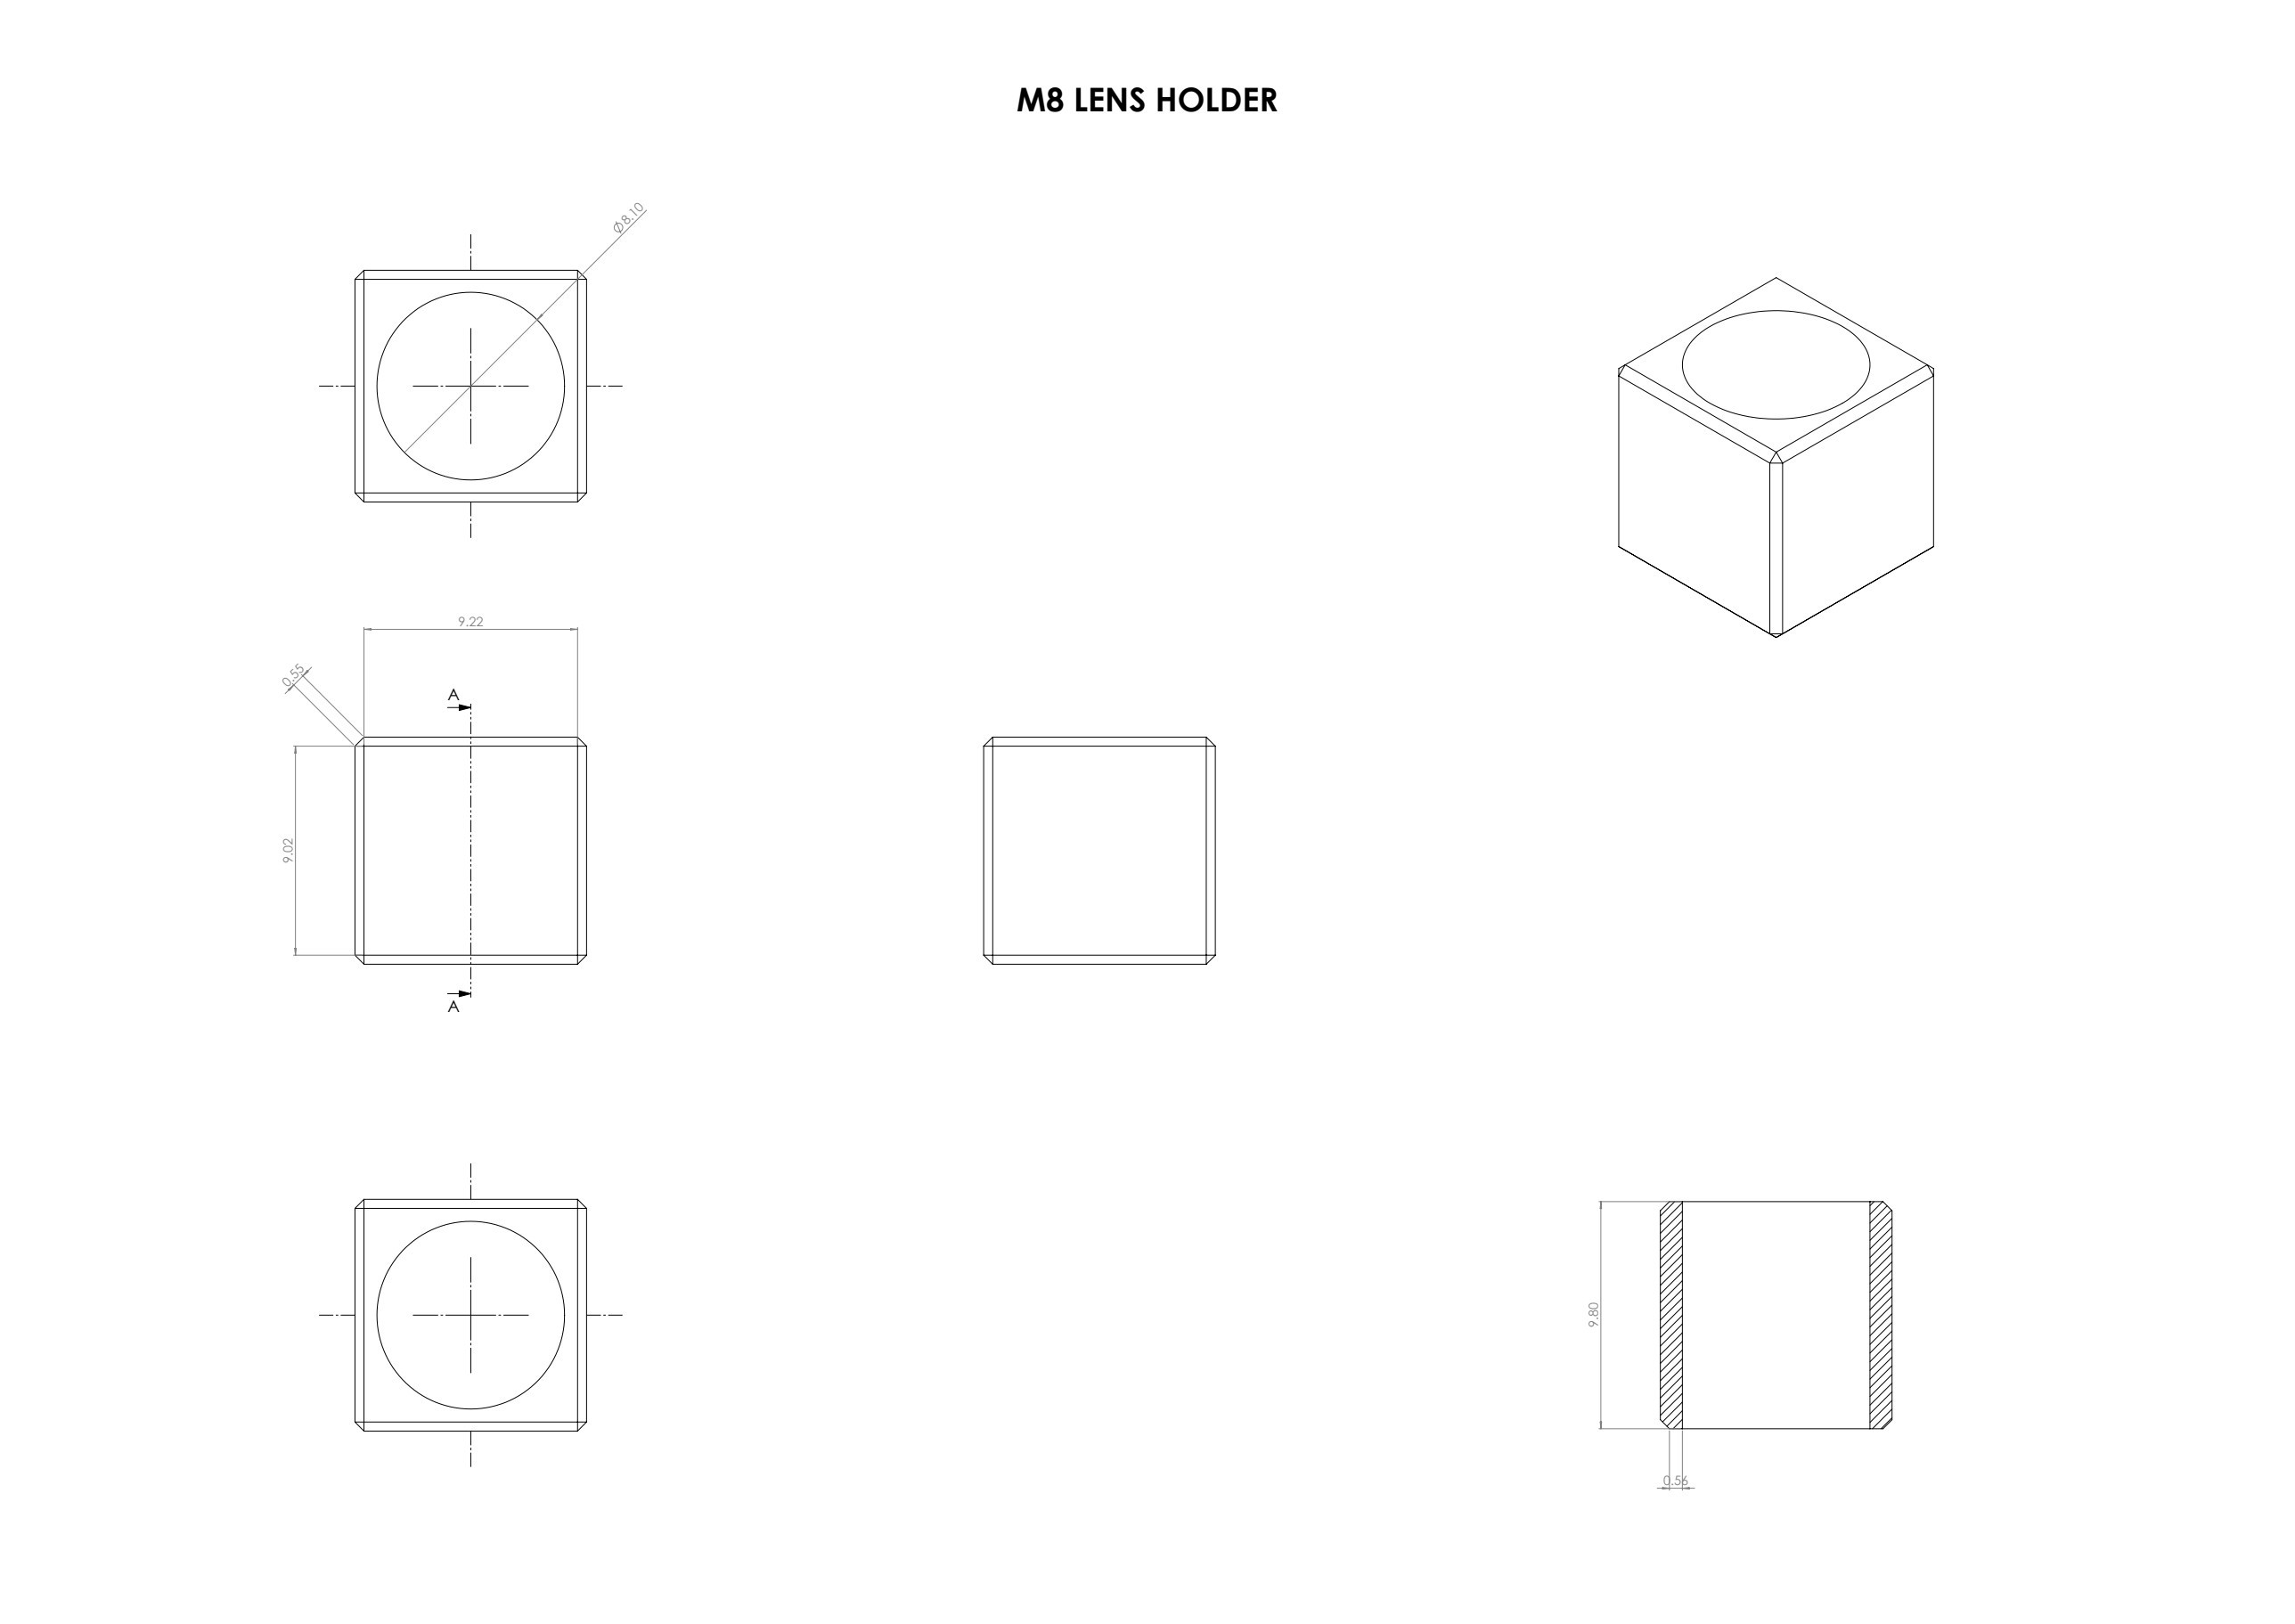
ISO-10303-21;
HEADER;
/* Generated by software containing ST-Developer
 * from STEP Tools, Inc. (www.steptools.com) 
 */

FILE_DESCRIPTION(
/* description */ (''),
/* implementation_level */ '2;1');

FILE_NAME(
/* name */ '06_M8_Lens_Holder.step',
/* time_stamp */ '2026-10-21T02:01:14-07:00',
/* author */ (''),
/* organization */ (''),
/* preprocessor_version */ 'ST-DEVELOPER v20.2',
/* originating_system */ 'Autodesk Translation Framework v15.15.0.0',
/* authorisation */ '');

FILE_SCHEMA (('AUTOMOTIVE_DESIGN { 1 0 10303 214 3 1 1 }'));
ENDSEC;

DATA;
#10=MECHANICAL_DESIGN_GEOMETRIC_PRESENTATION_REPRESENTATION('',(#619),#37181);
#593=SHAPE_REPRESENTATION_RELATIONSHIP('SRR','None',#37243,#606);
#606=ADVANCED_BREP_SHAPE_REPRESENTATION('',(#632),#37173);
#619=STYLED_ITEM('',(#37366),#632);
#632=MANIFOLD_SOLID_BREP('Body1',#14781);
#674=FACE_BOUND('',#2614,.T.);
#675=FACE_BOUND('',#2617,.T.);
#726=CYLINDRICAL_SURFACE('',#15454,4.05);
#1094=CIRCLE('',#15449,4.05);
#1095=CIRCLE('',#15452,4.05);
#1717=FACE_OUTER_BOUND('',#2591,.T.);
#1718=FACE_OUTER_BOUND('',#2592,.T.);
#1719=FACE_OUTER_BOUND('',#2593,.T.);
#1720=FACE_OUTER_BOUND('',#2594,.T.);
#1721=FACE_OUTER_BOUND('',#2595,.T.);
#1722=FACE_OUTER_BOUND('',#2596,.T.);
#1723=FACE_OUTER_BOUND('',#2597,.T.);
#1724=FACE_OUTER_BOUND('',#2598,.T.);
#1725=FACE_OUTER_BOUND('',#2599,.T.);
#1726=FACE_OUTER_BOUND('',#2600,.T.);
#1727=FACE_OUTER_BOUND('',#2601,.T.);
#1728=FACE_OUTER_BOUND('',#2602,.T.);
#1729=FACE_OUTER_BOUND('',#2603,.T.);
#1730=FACE_OUTER_BOUND('',#2604,.T.);
#1731=FACE_OUTER_BOUND('',#2605,.T.);
#1732=FACE_OUTER_BOUND('',#2606,.T.);
#1733=FACE_OUTER_BOUND('',#2607,.T.);
#1734=FACE_OUTER_BOUND('',#2608,.T.);
#1735=FACE_OUTER_BOUND('',#2609,.T.);
#1736=FACE_OUTER_BOUND('',#2610,.T.);
#1737=FACE_OUTER_BOUND('',#2611,.T.);
#1738=FACE_OUTER_BOUND('',#2612,.T.);
#1739=FACE_OUTER_BOUND('',#2613,.T.);
#1740=FACE_OUTER_BOUND('',#2615,.T.);
#1741=FACE_OUTER_BOUND('',#2616,.T.);
#1742=FACE_OUTER_BOUND('',#2618,.T.);
#1743=FACE_OUTER_BOUND('',#2619,.T.);
#2591=EDGE_LOOP('',(#10837,#10838,#10839));
#2592=EDGE_LOOP('',(#10840,#10841,#10842));
#2593=EDGE_LOOP('',(#10843,#10844,#10845));
#2594=EDGE_LOOP('',(#10846,#10847,#10848));
#2595=EDGE_LOOP('',(#10849,#10850,#10851));
#2596=EDGE_LOOP('',(#10852,#10853,#10854));
#2597=EDGE_LOOP('',(#10855,#10856,#10857));
#2598=EDGE_LOOP('',(#10858,#10859,#10860,#10861));
#2599=EDGE_LOOP('',(#10862,#10863,#10864));
#2600=EDGE_LOOP('',(#10865,#10866,#10867,#10868));
#2601=EDGE_LOOP('',(#10869,#10870,#10871,#10872));
#2602=EDGE_LOOP('',(#10873,#10874,#10875,#10876));
#2603=EDGE_LOOP('',(#10877,#10878,#10879,#10880));
#2604=EDGE_LOOP('',(#10881,#10882,#10883,#10884));
#2605=EDGE_LOOP('',(#10885,#10886,#10887,#10888));
#2606=EDGE_LOOP('',(#10889,#10890,#10891,#10892));
#2607=EDGE_LOOP('',(#10893,#10894,#10895,#10896));
#2608=EDGE_LOOP('',(#10897,#10898,#10899,#10900));
#2609=EDGE_LOOP('',(#10901,#10902,#10903,#10904));
#2610=EDGE_LOOP('',(#10905,#10906,#10907,#10908));
#2611=EDGE_LOOP('',(#10909,#10910,#10911,#10912));
#2612=EDGE_LOOP('',(#10913,#10914,#10915,#10916));
#2613=EDGE_LOOP('',(#10917,#10918,#10919,#10920));
#2614=EDGE_LOOP('',(#10921));
#2615=EDGE_LOOP('',(#10922,#10923,#10924,#10925));
#2616=EDGE_LOOP('',(#10926,#10927,#10928,#10929));
#2617=EDGE_LOOP('',(#10930));
#2618=EDGE_LOOP('',(#10931,#10932,#10933,#10934));
#2619=EDGE_LOOP('',(#10935,#10936,#10937,#10938));
#3832=LINE('',#21697,#5071);
#3833=LINE('',#21699,#5072);
#3834=LINE('',#21700,#5073);
#3835=LINE('',#21704,#5074);
#3836=LINE('',#21706,#5075);
#3837=LINE('',#21707,#5076);
#3838=LINE('',#21711,#5077);
#3839=LINE('',#21713,#5078);
#3840=LINE('',#21714,#5079);
#3841=LINE('',#21718,#5080);
#3842=LINE('',#21720,#5081);
#3843=LINE('',#21721,#5082);
#3844=LINE('',#21725,#5083);
#3845=LINE('',#21727,#5084);
#3846=LINE('',#21728,#5085);
#3847=LINE('',#21732,#5086);
#3848=LINE('',#21734,#5087);
#3849=LINE('',#21735,#5088);
#3850=LINE('',#21739,#5089);
#3851=LINE('',#21741,#5090);
#3852=LINE('',#21742,#5091);
#3853=LINE('',#21744,#5092);
#3854=LINE('',#21745,#5093);
#3855=LINE('',#21749,#5094);
#3856=LINE('',#21751,#5095);
#3857=LINE('',#21752,#5096);
#3858=LINE('',#21754,#5097);
#3859=LINE('',#21755,#5098);
#3860=LINE('',#21757,#5099);
#3861=LINE('',#21758,#5100);
#3862=LINE('',#21760,#5101);
#3863=LINE('',#21761,#5102);
#3864=LINE('',#21763,#5103);
#3865=LINE('',#21764,#5104);
#3866=LINE('',#21766,#5105);
#3867=LINE('',#21767,#5106);
#3868=LINE('',#21769,#5107);
#3869=LINE('',#21770,#5108);
#3870=LINE('',#21772,#5109);
#3871=LINE('',#21773,#5110);
#3872=LINE('',#21775,#5111);
#3873=LINE('',#21776,#5112);
#3874=LINE('',#21778,#5113);
#3875=LINE('',#21779,#5114);
#3876=LINE('',#21781,#5115);
#3877=LINE('',#21782,#5116);
#3878=LINE('',#21784,#5117);
#3879=LINE('',#21785,#5118);
#3880=LINE('',#21797,#5119);
#5071=VECTOR('',#17742,10.);
#5072=VECTOR('',#17743,10.);
#5073=VECTOR('',#17744,10.);
#5074=VECTOR('',#17747,10.);
#5075=VECTOR('',#17748,10.);
#5076=VECTOR('',#17749,10.);
#5077=VECTOR('',#17752,10.);
#5078=VECTOR('',#17753,10.);
#5079=VECTOR('',#17754,10.);
#5080=VECTOR('',#17757,10.);
#5081=VECTOR('',#17758,10.);
#5082=VECTOR('',#17759,10.);
#5083=VECTOR('',#17762,10.);
#5084=VECTOR('',#17763,10.);
#5085=VECTOR('',#17764,10.);
#5086=VECTOR('',#17767,10.);
#5087=VECTOR('',#17768,10.);
#5088=VECTOR('',#17769,10.);
#5089=VECTOR('',#17772,10.);
#5090=VECTOR('',#17773,10.);
#5091=VECTOR('',#17774,10.);
#5092=VECTOR('',#17777,10.);
#5093=VECTOR('',#17778,10.);
#5094=VECTOR('',#17781,10.);
#5095=VECTOR('',#17782,10.);
#5096=VECTOR('',#17783,10.);
#5097=VECTOR('',#17786,10.);
#5098=VECTOR('',#17787,10.);
#5099=VECTOR('',#17790,10.);
#5100=VECTOR('',#17791,10.);
#5101=VECTOR('',#17794,10.);
#5102=VECTOR('',#17795,10.);
#5103=VECTOR('',#17798,10.);
#5104=VECTOR('',#17799,10.);
#5105=VECTOR('',#17802,10.);
#5106=VECTOR('',#17803,10.);
#5107=VECTOR('',#17806,10.);
#5108=VECTOR('',#17807,10.);
#5109=VECTOR('',#17810,10.);
#5110=VECTOR('',#17811,10.);
#5111=VECTOR('',#17814,10.);
#5112=VECTOR('',#17815,10.);
#5113=VECTOR('',#17818,10.);
#5114=VECTOR('',#17819,10.);
#5115=VECTOR('',#17822,10.);
#5116=VECTOR('',#17823,10.);
#5117=VECTOR('',#17826,10.);
#5118=VECTOR('',#17827,10.);
#5119=VECTOR('',#17846,4.05);
#6183=VERTEX_POINT('',#21695);
#6184=VERTEX_POINT('',#21696);
#6185=VERTEX_POINT('',#21698);
#6186=VERTEX_POINT('',#21702);
#6187=VERTEX_POINT('',#21703);
#6188=VERTEX_POINT('',#21705);
#6189=VERTEX_POINT('',#21709);
#6190=VERTEX_POINT('',#21710);
#6191=VERTEX_POINT('',#21712);
#6192=VERTEX_POINT('',#21716);
#6193=VERTEX_POINT('',#21717);
#6194=VERTEX_POINT('',#21719);
#6195=VERTEX_POINT('',#21723);
#6196=VERTEX_POINT('',#21724);
#6197=VERTEX_POINT('',#21726);
#6198=VERTEX_POINT('',#21730);
#6199=VERTEX_POINT('',#21731);
#6200=VERTEX_POINT('',#21733);
#6201=VERTEX_POINT('',#21737);
#6202=VERTEX_POINT('',#21738);
#6203=VERTEX_POINT('',#21740);
#6204=VERTEX_POINT('',#21747);
#6205=VERTEX_POINT('',#21748);
#6206=VERTEX_POINT('',#21750);
#6207=VERTEX_POINT('',#21789);
#6208=VERTEX_POINT('',#21793);
#7860=EDGE_CURVE('',#6183,#6184,#3832,.T.);
#7861=EDGE_CURVE('',#6185,#6183,#3833,.T.);
#7862=EDGE_CURVE('',#6184,#6185,#3834,.T.);
#7863=EDGE_CURVE('',#6186,#6187,#3835,.T.);
#7864=EDGE_CURVE('',#6188,#6186,#3836,.T.);
#7865=EDGE_CURVE('',#6187,#6188,#3837,.T.);
#7866=EDGE_CURVE('',#6189,#6190,#3838,.T.);
#7867=EDGE_CURVE('',#6191,#6189,#3839,.T.);
#7868=EDGE_CURVE('',#6190,#6191,#3840,.T.);
#7869=EDGE_CURVE('',#6192,#6193,#3841,.T.);
#7870=EDGE_CURVE('',#6194,#6192,#3842,.T.);
#7871=EDGE_CURVE('',#6193,#6194,#3843,.T.);
#7872=EDGE_CURVE('',#6195,#6196,#3844,.T.);
#7873=EDGE_CURVE('',#6197,#6195,#3845,.T.);
#7874=EDGE_CURVE('',#6196,#6197,#3846,.T.);
#7875=EDGE_CURVE('',#6198,#6199,#3847,.T.);
#7876=EDGE_CURVE('',#6200,#6198,#3848,.T.);
#7877=EDGE_CURVE('',#6199,#6200,#3849,.T.);
#7878=EDGE_CURVE('',#6201,#6202,#3850,.T.);
#7879=EDGE_CURVE('',#6203,#6201,#3851,.T.);
#7880=EDGE_CURVE('',#6202,#6203,#3852,.T.);
#7881=EDGE_CURVE('',#6191,#6203,#3853,.T.);
#7882=EDGE_CURVE('',#6201,#6190,#3854,.T.);
#7883=EDGE_CURVE('',#6204,#6205,#3855,.T.);
#7884=EDGE_CURVE('',#6206,#6204,#3856,.T.);
#7885=EDGE_CURVE('',#6205,#6206,#3857,.T.);
#7886=EDGE_CURVE('',#6204,#6197,#3858,.T.);
#7887=EDGE_CURVE('',#6195,#6206,#3859,.T.);
#7888=EDGE_CURVE('',#6198,#6205,#3860,.T.);
#7889=EDGE_CURVE('',#6206,#6200,#3861,.T.);
#7890=EDGE_CURVE('',#6203,#6204,#3862,.T.);
#7891=EDGE_CURVE('',#6205,#6202,#3863,.T.);
#7892=EDGE_CURVE('',#6192,#6201,#3864,.T.);
#7893=EDGE_CURVE('',#6202,#6194,#3865,.T.);
#7894=EDGE_CURVE('',#6187,#6199,#3866,.T.);
#7895=EDGE_CURVE('',#6200,#6186,#3867,.T.);
#7896=EDGE_CURVE('',#6199,#6193,#3868,.T.);
#7897=EDGE_CURVE('',#6194,#6198,#3869,.T.);
#7898=EDGE_CURVE('',#6197,#6191,#3870,.T.);
#7899=EDGE_CURVE('',#6189,#6196,#3871,.T.);
#7900=EDGE_CURVE('',#6186,#6195,#3872,.T.);
#7901=EDGE_CURVE('',#6196,#6188,#3873,.T.);
#7902=EDGE_CURVE('',#6193,#6184,#3874,.T.);
#7903=EDGE_CURVE('',#6185,#6192,#3875,.T.);
#7904=EDGE_CURVE('',#6183,#6189,#3876,.T.);
#7905=EDGE_CURVE('',#6190,#6185,#3877,.T.);
#7906=EDGE_CURVE('',#6184,#6187,#3878,.T.);
#7907=EDGE_CURVE('',#6188,#6183,#3879,.T.);
#7908=EDGE_CURVE('',#6207,#6207,#1094,.T.);
#7909=EDGE_CURVE('',#6208,#6208,#1095,.T.);
#7910=EDGE_CURVE('',#6208,#6207,#3880,.T.);
#10837=ORIENTED_EDGE('',*,*,#7860,.F.);
#10838=ORIENTED_EDGE('',*,*,#7861,.F.);
#10839=ORIENTED_EDGE('',*,*,#7862,.F.);
#10840=ORIENTED_EDGE('',*,*,#7863,.F.);
#10841=ORIENTED_EDGE('',*,*,#7864,.F.);
#10842=ORIENTED_EDGE('',*,*,#7865,.F.);
#10843=ORIENTED_EDGE('',*,*,#7866,.F.);
#10844=ORIENTED_EDGE('',*,*,#7867,.F.);
#10845=ORIENTED_EDGE('',*,*,#7868,.F.);
#10846=ORIENTED_EDGE('',*,*,#7869,.F.);
#10847=ORIENTED_EDGE('',*,*,#7870,.F.);
#10848=ORIENTED_EDGE('',*,*,#7871,.F.);
#10849=ORIENTED_EDGE('',*,*,#7872,.F.);
#10850=ORIENTED_EDGE('',*,*,#7873,.F.);
#10851=ORIENTED_EDGE('',*,*,#7874,.F.);
#10852=ORIENTED_EDGE('',*,*,#7875,.F.);
#10853=ORIENTED_EDGE('',*,*,#7876,.F.);
#10854=ORIENTED_EDGE('',*,*,#7877,.F.);
#10855=ORIENTED_EDGE('',*,*,#7878,.F.);
#10856=ORIENTED_EDGE('',*,*,#7879,.F.);
#10857=ORIENTED_EDGE('',*,*,#7880,.F.);
#10858=ORIENTED_EDGE('',*,*,#7868,.T.);
#10859=ORIENTED_EDGE('',*,*,#7881,.T.);
#10860=ORIENTED_EDGE('',*,*,#7879,.T.);
#10861=ORIENTED_EDGE('',*,*,#7882,.T.);
#10862=ORIENTED_EDGE('',*,*,#7883,.F.);
#10863=ORIENTED_EDGE('',*,*,#7884,.F.);
#10864=ORIENTED_EDGE('',*,*,#7885,.F.);
#10865=ORIENTED_EDGE('',*,*,#7884,.T.);
#10866=ORIENTED_EDGE('',*,*,#7886,.T.);
#10867=ORIENTED_EDGE('',*,*,#7873,.T.);
#10868=ORIENTED_EDGE('',*,*,#7887,.T.);
#10869=ORIENTED_EDGE('',*,*,#7876,.T.);
#10870=ORIENTED_EDGE('',*,*,#7888,.T.);
#10871=ORIENTED_EDGE('',*,*,#7885,.T.);
#10872=ORIENTED_EDGE('',*,*,#7889,.T.);
#10873=ORIENTED_EDGE('',*,*,#7880,.T.);
#10874=ORIENTED_EDGE('',*,*,#7890,.T.);
#10875=ORIENTED_EDGE('',*,*,#7883,.T.);
#10876=ORIENTED_EDGE('',*,*,#7891,.T.);
#10877=ORIENTED_EDGE('',*,*,#7870,.T.);
#10878=ORIENTED_EDGE('',*,*,#7892,.T.);
#10879=ORIENTED_EDGE('',*,*,#7878,.T.);
#10880=ORIENTED_EDGE('',*,*,#7893,.T.);
#10881=ORIENTED_EDGE('',*,*,#7863,.T.);
#10882=ORIENTED_EDGE('',*,*,#7894,.T.);
#10883=ORIENTED_EDGE('',*,*,#7877,.T.);
#10884=ORIENTED_EDGE('',*,*,#7895,.T.);
#10885=ORIENTED_EDGE('',*,*,#7875,.T.);
#10886=ORIENTED_EDGE('',*,*,#7896,.T.);
#10887=ORIENTED_EDGE('',*,*,#7871,.T.);
#10888=ORIENTED_EDGE('',*,*,#7897,.T.);
#10889=ORIENTED_EDGE('',*,*,#7874,.T.);
#10890=ORIENTED_EDGE('',*,*,#7898,.T.);
#10891=ORIENTED_EDGE('',*,*,#7867,.T.);
#10892=ORIENTED_EDGE('',*,*,#7899,.T.);
#10893=ORIENTED_EDGE('',*,*,#7864,.T.);
#10894=ORIENTED_EDGE('',*,*,#7900,.T.);
#10895=ORIENTED_EDGE('',*,*,#7872,.T.);
#10896=ORIENTED_EDGE('',*,*,#7901,.T.);
#10897=ORIENTED_EDGE('',*,*,#7869,.T.);
#10898=ORIENTED_EDGE('',*,*,#7902,.T.);
#10899=ORIENTED_EDGE('',*,*,#7862,.T.);
#10900=ORIENTED_EDGE('',*,*,#7903,.T.);
#10901=ORIENTED_EDGE('',*,*,#7861,.T.);
#10902=ORIENTED_EDGE('',*,*,#7904,.T.);
#10903=ORIENTED_EDGE('',*,*,#7866,.T.);
#10904=ORIENTED_EDGE('',*,*,#7905,.T.);
#10905=ORIENTED_EDGE('',*,*,#7860,.T.);
#10906=ORIENTED_EDGE('',*,*,#7906,.T.);
#10907=ORIENTED_EDGE('',*,*,#7865,.T.);
#10908=ORIENTED_EDGE('',*,*,#7907,.T.);
#10909=ORIENTED_EDGE('',*,*,#7882,.F.);
#10910=ORIENTED_EDGE('',*,*,#7892,.F.);
#10911=ORIENTED_EDGE('',*,*,#7903,.F.);
#10912=ORIENTED_EDGE('',*,*,#7905,.F.);
#10913=ORIENTED_EDGE('',*,*,#7887,.F.);
#10914=ORIENTED_EDGE('',*,*,#7900,.F.);
#10915=ORIENTED_EDGE('',*,*,#7895,.F.);
#10916=ORIENTED_EDGE('',*,*,#7889,.F.);
#10917=ORIENTED_EDGE('',*,*,#7886,.F.);
#10918=ORIENTED_EDGE('',*,*,#7890,.F.);
#10919=ORIENTED_EDGE('',*,*,#7881,.F.);
#10920=ORIENTED_EDGE('',*,*,#7898,.F.);
#10921=ORIENTED_EDGE('',*,*,#7908,.T.);
#10922=ORIENTED_EDGE('',*,*,#7888,.F.);
#10923=ORIENTED_EDGE('',*,*,#7897,.F.);
#10924=ORIENTED_EDGE('',*,*,#7893,.F.);
#10925=ORIENTED_EDGE('',*,*,#7891,.F.);
#10926=ORIENTED_EDGE('',*,*,#7894,.F.);
#10927=ORIENTED_EDGE('',*,*,#7906,.F.);
#10928=ORIENTED_EDGE('',*,*,#7902,.F.);
#10929=ORIENTED_EDGE('',*,*,#7896,.F.);
#10930=ORIENTED_EDGE('',*,*,#7909,.T.);
#10931=ORIENTED_EDGE('',*,*,#7899,.F.);
#10932=ORIENTED_EDGE('',*,*,#7904,.F.);
#10933=ORIENTED_EDGE('',*,*,#7907,.F.);
#10934=ORIENTED_EDGE('',*,*,#7901,.F.);
#10935=ORIENTED_EDGE('',*,*,#7909,.F.);
#10936=ORIENTED_EDGE('',*,*,#7910,.T.);
#10937=ORIENTED_EDGE('',*,*,#7908,.F.);
#10938=ORIENTED_EDGE('',*,*,#7910,.F.);
#13700=PLANE('',#15426);
#13701=PLANE('',#15427);
#13702=PLANE('',#15428);
#13703=PLANE('',#15429);
#13704=PLANE('',#15430);
#13705=PLANE('',#15431);
#13706=PLANE('',#15432);
#13707=PLANE('',#15433);
#13708=PLANE('',#15434);
#13709=PLANE('',#15435);
#13710=PLANE('',#15436);
#13711=PLANE('',#15437);
#13712=PLANE('',#15438);
#13713=PLANE('',#15439);
#13714=PLANE('',#15440);
#13715=PLANE('',#15441);
#13716=PLANE('',#15442);
#13717=PLANE('',#15443);
#13718=PLANE('',#15444);
#13719=PLANE('',#15445);
#13720=PLANE('',#15446);
#13721=PLANE('',#15447);
#13722=PLANE('',#15448);
#13723=PLANE('',#15450);
#13724=PLANE('',#15451);
#13725=PLANE('',#15453);
#14285=ADVANCED_FACE('',(#1717),#13700,.T.);
#14286=ADVANCED_FACE('',(#1718),#13701,.T.);
#14287=ADVANCED_FACE('',(#1719),#13702,.T.);
#14288=ADVANCED_FACE('',(#1720),#13703,.T.);
#14289=ADVANCED_FACE('',(#1721),#13704,.T.);
#14290=ADVANCED_FACE('',(#1722),#13705,.T.);
#14291=ADVANCED_FACE('',(#1723),#13706,.T.);
#14292=ADVANCED_FACE('',(#1724),#13707,.T.);
#14293=ADVANCED_FACE('',(#1725),#13708,.T.);
#14294=ADVANCED_FACE('',(#1726),#13709,.T.);
#14295=ADVANCED_FACE('',(#1727),#13710,.T.);
#14296=ADVANCED_FACE('',(#1728),#13711,.T.);
#14297=ADVANCED_FACE('',(#1729),#13712,.T.);
#14298=ADVANCED_FACE('',(#1730),#13713,.T.);
#14299=ADVANCED_FACE('',(#1731),#13714,.T.);
#14300=ADVANCED_FACE('',(#1732),#13715,.T.);
#14301=ADVANCED_FACE('',(#1733),#13716,.T.);
#14302=ADVANCED_FACE('',(#1734),#13717,.T.);
#14303=ADVANCED_FACE('',(#1735),#13718,.T.);
#14304=ADVANCED_FACE('',(#1736),#13719,.T.);
#14305=ADVANCED_FACE('',(#1737),#13720,.T.);
#14306=ADVANCED_FACE('',(#1738),#13721,.T.);
#14307=ADVANCED_FACE('',(#1739,#674),#13722,.F.);
#14308=ADVANCED_FACE('',(#1740),#13723,.T.);
#14309=ADVANCED_FACE('',(#1741,#675),#13724,.T.);
#14310=ADVANCED_FACE('',(#1742),#13725,.T.);
#14311=ADVANCED_FACE('',(#1743),#726,.F.);
#14781=CLOSED_SHELL('',(#14285,#14286,#14287,#14288,#14289,#14290,#14291,
#14292,#14293,#14294,#14295,#14296,#14297,#14298,#14299,#14300,#14301,#14302,
#14303,#14304,#14305,#14306,#14307,#14308,#14309,#14310,#14311));
#15425=AXIS2_PLACEMENT_3D('',#21693,#17738,#17739);
#15426=AXIS2_PLACEMENT_3D('',#21694,#17740,#17741);
#15427=AXIS2_PLACEMENT_3D('',#21701,#17745,#17746);
#15428=AXIS2_PLACEMENT_3D('',#21708,#17750,#17751);
#15429=AXIS2_PLACEMENT_3D('',#21715,#17755,#17756);
#15430=AXIS2_PLACEMENT_3D('',#21722,#17760,#17761);
#15431=AXIS2_PLACEMENT_3D('',#21729,#17765,#17766);
#15432=AXIS2_PLACEMENT_3D('',#21736,#17770,#17771);
#15433=AXIS2_PLACEMENT_3D('',#21743,#17775,#17776);
#15434=AXIS2_PLACEMENT_3D('',#21746,#17779,#17780);
#15435=AXIS2_PLACEMENT_3D('',#21753,#17784,#17785);
#15436=AXIS2_PLACEMENT_3D('',#21756,#17788,#17789);
#15437=AXIS2_PLACEMENT_3D('',#21759,#17792,#17793);
#15438=AXIS2_PLACEMENT_3D('',#21762,#17796,#17797);
#15439=AXIS2_PLACEMENT_3D('',#21765,#17800,#17801);
#15440=AXIS2_PLACEMENT_3D('',#21768,#17804,#17805);
#15441=AXIS2_PLACEMENT_3D('',#21771,#17808,#17809);
#15442=AXIS2_PLACEMENT_3D('',#21774,#17812,#17813);
#15443=AXIS2_PLACEMENT_3D('',#21777,#17816,#17817);
#15444=AXIS2_PLACEMENT_3D('',#21780,#17820,#17821);
#15445=AXIS2_PLACEMENT_3D('',#21783,#17824,#17825);
#15446=AXIS2_PLACEMENT_3D('',#21786,#17828,#17829);
#15447=AXIS2_PLACEMENT_3D('',#21787,#17830,#17831);
#15448=AXIS2_PLACEMENT_3D('',#21788,#17832,#17833);
#15449=AXIS2_PLACEMENT_3D('',#21790,#17834,#17835);
#15450=AXIS2_PLACEMENT_3D('',#21791,#17836,#17837);
#15451=AXIS2_PLACEMENT_3D('',#21792,#17838,#17839);
#15452=AXIS2_PLACEMENT_3D('',#21794,#17840,#17841);
#15453=AXIS2_PLACEMENT_3D('',#21795,#17842,#17843);
#15454=AXIS2_PLACEMENT_3D('',#21796,#17844,#17845);
#17738=DIRECTION('axis',(0.,0.,1.));
#17739=DIRECTION('refdir',(1.,0.,0.));
#17740=DIRECTION('center_axis',(0.577350269189623,0.577350269189625,-0.57735026918963));
#17741=DIRECTION('ref_axis',(-0.707106781186552,0.,-0.707106781186544));
#17742=DIRECTION('',(-0.707106781186548,0.707106781186546,0.));
#17743=DIRECTION('',(0.707106781186552,0.,0.707106781186543));
#17744=DIRECTION('',(0.,-0.70710678118655,-0.707106781186544));
#17745=DIRECTION('center_axis',(0.577350269189623,0.577350269189625,0.57735026918963));
#17746=DIRECTION('ref_axis',(0.707106781186552,0.,-0.707106781186543));
#17747=DIRECTION('',(0.,0.70710678118655,-0.707106781186544));
#17748=DIRECTION('',(-0.707106781186552,0.,0.707106781186543));
#17749=DIRECTION('',(0.707106781186548,-0.707106781186546,0.));
#17750=DIRECTION('center_axis',(0.577350269189624,-0.577350269189624,-0.57735026918963));
#17751=DIRECTION('ref_axis',(-0.707106781186552,0.,-0.707106781186544));
#17752=DIRECTION('',(-0.707106781186552,0.,-0.707106781186543));
#17753=DIRECTION('',(0.707106781186547,0.707106781186547,0.));
#17754=DIRECTION('',(0.,-0.707106781186552,0.707106781186543));
#17755=DIRECTION('center_axis',(-0.577350269189625,0.577350269189624,-0.577350269189629));
#17756=DIRECTION('ref_axis',(-0.70710678118655,0.,0.707106781186545));
#17757=DIRECTION('',(0.,0.70710678118655,0.707106781186544));
#17758=DIRECTION('',(0.70710678118655,0.,-0.707106781186545));
#17759=DIRECTION('',(-0.707106781186546,-0.707106781186549,0.));
#17760=DIRECTION('center_axis',(0.577350269189624,-0.577350269189624,0.57735026918963));
#17761=DIRECTION('ref_axis',(0.707106781186552,0.,-0.707106781186544));
#17762=DIRECTION('',(0.707106781186552,0.,-0.707106781186543));
#17763=DIRECTION('',(0.,0.707106781186552,0.707106781186543));
#17764=DIRECTION('',(-0.707106781186547,-0.707106781186547,0.));
#17765=DIRECTION('center_axis',(-0.577350269189626,0.577350269189625,0.577350269189626));
#17766=DIRECTION('ref_axis',(0.707106781186547,0.,0.707106781186547));
#17767=DIRECTION('',(0.707106781186546,0.707106781186549,0.));
#17768=DIRECTION('',(-0.707106781186547,0.,-0.707106781186547));
#17769=DIRECTION('',(-4.02587809918918E-15,-0.70710678118655,0.707106781186544));
#17770=DIRECTION('center_axis',(-0.577350269189626,-0.577350269189623,-0.577350269189629));
#17771=DIRECTION('ref_axis',(-0.70710678118655,0.,0.707106781186545));
#17772=DIRECTION('',(-0.70710678118655,0.,0.707106781186545));
#17773=DIRECTION('',(0.,0.707106781186552,-0.707106781186543));
#17774=DIRECTION('',(0.707106781186545,-0.70710678118655,0.));
#17775=DIRECTION('center_axis',(0.,-0.707106781186543,-0.707106781186552));
#17776=DIRECTION('ref_axis',(-1.,0.,0.));
#17777=DIRECTION('',(-1.,0.,0.));
#17778=DIRECTION('',(1.,0.,0.));
#17779=DIRECTION('center_axis',(-0.577350269189627,-0.577350269189624,0.577350269189627));
#17780=DIRECTION('ref_axis',(0.707106781186547,0.,0.707106781186547));
#17781=DIRECTION('',(-0.707106781186545,0.70710678118655,0.));
#17782=DIRECTION('',(4.02587809918917E-15,-0.707106781186552,-0.707106781186543));
#17783=DIRECTION('',(0.707106781186547,0.,0.707106781186547));
#17784=DIRECTION('center_axis',(0.,-0.707106781186543,0.707106781186552));
#17785=DIRECTION('ref_axis',(1.,0.,0.));
#17786=DIRECTION('',(1.,0.,0.));
#17787=DIRECTION('',(-1.,0.,0.));
#17788=DIRECTION('center_axis',(-0.707106781186548,0.,0.707106781186548));
#17789=DIRECTION('ref_axis',(0.707106781186548,0.,0.707106781186548));
#17790=DIRECTION('',(0.,-1.,0.));
#17791=DIRECTION('',(0.,1.,0.));
#17792=DIRECTION('center_axis',(-0.70710678118655,-0.707106781186546,0.));
#17793=DIRECTION('ref_axis',(0.,0.,1.));
#17794=DIRECTION('',(0.,0.,1.));
#17795=DIRECTION('',(0.,0.,-1.));
#17796=DIRECTION('center_axis',(-0.707106781186545,0.,-0.70710678118655));
#17797=DIRECTION('ref_axis',(-0.70710678118655,0.,0.707106781186545));
#17798=DIRECTION('',(0.,-1.,0.));
#17799=DIRECTION('',(0.,1.,0.));
#17800=DIRECTION('center_axis',(0.,0.707106781186545,0.707106781186551));
#17801=DIRECTION('ref_axis',(1.,0.,0.));
#17802=DIRECTION('',(-1.,0.,0.));
#17803=DIRECTION('',(1.,0.,0.));
#17804=DIRECTION('center_axis',(-0.707106781186549,0.707106781186546,0.));
#17805=DIRECTION('ref_axis',(0.,0.,1.));
#17806=DIRECTION('',(0.,0.,-1.));
#17807=DIRECTION('',(0.,0.,1.));
#17808=DIRECTION('center_axis',(0.707106781186548,-0.707106781186548,0.));
#17809=DIRECTION('ref_axis',(0.,0.,-1.));
#17810=DIRECTION('',(0.,0.,-1.));
#17811=DIRECTION('',(0.,0.,1.));
#17812=DIRECTION('center_axis',(0.707106781186543,0.,0.707106781186552));
#17813=DIRECTION('ref_axis',(0.707106781186552,0.,-0.707106781186543));
#17814=DIRECTION('',(0.,-1.,0.));
#17815=DIRECTION('',(0.,1.,0.));
#17816=DIRECTION('center_axis',(0.,0.707106781186545,-0.707106781186551));
#17817=DIRECTION('ref_axis',(-1.,0.,0.));
#17818=DIRECTION('',(1.,0.,0.));
#17819=DIRECTION('',(-1.,0.,0.));
#17820=DIRECTION('center_axis',(0.707106781186543,0.,-0.707106781186552));
#17821=DIRECTION('ref_axis',(-0.707106781186552,0.,-0.707106781186543));
#17822=DIRECTION('',(0.,-1.,0.));
#17823=DIRECTION('',(0.,1.,0.));
#17824=DIRECTION('center_axis',(0.707106781186547,0.707106781186549,0.));
#17825=DIRECTION('ref_axis',(0.,0.,-1.));
#17826=DIRECTION('',(0.,0.,1.));
#17827=DIRECTION('',(0.,0.,-1.));
#17828=DIRECTION('center_axis',(0.,0.,-1.));
#17829=DIRECTION('ref_axis',(-1.,0.,0.));
#17830=DIRECTION('center_axis',(0.,0.,1.));
#17831=DIRECTION('ref_axis',(1.,0.,0.));
#17832=DIRECTION('center_axis',(0.,1.,0.));
#17833=DIRECTION('ref_axis',(1.,0.,0.));
#17834=DIRECTION('center_axis',(0.,1.,0.));
#17835=DIRECTION('ref_axis',(1.,0.,0.));
#17836=DIRECTION('center_axis',(-1.,0.,0.));
#17837=DIRECTION('ref_axis',(0.,0.,1.));
#17838=DIRECTION('center_axis',(0.,1.,0.));
#17839=DIRECTION('ref_axis',(0.,0.,1.));
#17840=DIRECTION('center_axis',(0.,-1.,0.));
#17841=DIRECTION('ref_axis',(1.,0.,0.));
#17842=DIRECTION('center_axis',(1.,0.,0.));
#17843=DIRECTION('ref_axis',(0.,0.,-1.));
#17844=DIRECTION('center_axis',(0.,-1.,0.));
#17845=DIRECTION('ref_axis',(1.,0.,0.));
#17846=DIRECTION('',(0.,-1.,0.));
#21693=CARTESIAN_POINT('',(0.,0.,0.));
#21694=CARTESIAN_POINT('Origin',(28.61,1.61,-52.5));
#21695=CARTESIAN_POINT('',(29.,1.61,-52.11));
#21696=CARTESIAN_POINT('',(28.61,2.,-52.11));
#21697=CARTESIAN_POINT('',(29.,1.61,-52.11));
#21698=CARTESIAN_POINT('',(28.61,1.61,-52.5));
#21699=CARTESIAN_POINT('',(28.61,1.61,-52.5));
#21700=CARTESIAN_POINT('',(28.61,2.,-52.11));
#21701=CARTESIAN_POINT('Origin',(29.,1.61,-42.89));
#21702=CARTESIAN_POINT('',(28.61,1.61,-42.5));
#21703=CARTESIAN_POINT('',(28.61,2.,-42.89));
#21704=CARTESIAN_POINT('',(28.61,1.61,-42.5));
#21705=CARTESIAN_POINT('',(29.,1.61,-42.89));
#21706=CARTESIAN_POINT('',(29.,1.61,-42.89));
#21707=CARTESIAN_POINT('',(28.61,2.,-42.89));
#21708=CARTESIAN_POINT('Origin',(28.61,-7.8,-52.11));
#21709=CARTESIAN_POINT('',(29.,-7.41,-52.11));
#21710=CARTESIAN_POINT('',(28.61,-7.41,-52.5));
#21711=CARTESIAN_POINT('',(29.,-7.41,-52.11));
#21712=CARTESIAN_POINT('',(28.61,-7.8,-52.11));
#21713=CARTESIAN_POINT('',(28.61,-7.8,-52.11));
#21714=CARTESIAN_POINT('',(28.61,-7.41,-52.5));
#21715=CARTESIAN_POINT('Origin',(19.,1.61,-52.11));
#21716=CARTESIAN_POINT('',(19.39,1.61,-52.5));
#21717=CARTESIAN_POINT('',(19.39,2.,-52.11));
#21718=CARTESIAN_POINT('',(19.39,1.61,-52.5));
#21719=CARTESIAN_POINT('',(19.,1.61,-52.11));
#21720=CARTESIAN_POINT('',(19.,1.61,-52.11));
#21721=CARTESIAN_POINT('',(19.39,2.,-52.11));
#21722=CARTESIAN_POINT('Origin',(28.61,-7.8,-42.89));
#21723=CARTESIAN_POINT('',(28.61,-7.41,-42.5));
#21724=CARTESIAN_POINT('',(29.,-7.41,-42.89));
#21725=CARTESIAN_POINT('',(28.61,-7.41,-42.5));
#21726=CARTESIAN_POINT('',(28.61,-7.8,-42.89));
#21727=CARTESIAN_POINT('',(28.61,-7.8,-42.89));
#21728=CARTESIAN_POINT('',(29.,-7.41,-42.89));
#21729=CARTESIAN_POINT('Origin',(19.39,1.61,-42.5));
#21730=CARTESIAN_POINT('',(19.,1.61,-42.89));
#21731=CARTESIAN_POINT('',(19.39,2.,-42.89));
#21732=CARTESIAN_POINT('',(19.,1.61,-42.89));
#21733=CARTESIAN_POINT('',(19.39,1.61,-42.5));
#21734=CARTESIAN_POINT('',(19.39,1.61,-42.5));
#21735=CARTESIAN_POINT('',(19.39,2.,-42.89));
#21736=CARTESIAN_POINT('Origin',(19.39,-7.8,-52.11));
#21737=CARTESIAN_POINT('',(19.39,-7.41,-52.5));
#21738=CARTESIAN_POINT('',(19.,-7.41,-52.11));
#21739=CARTESIAN_POINT('',(19.39,-7.41,-52.5));
#21740=CARTESIAN_POINT('',(19.39,-7.8,-52.11));
#21741=CARTESIAN_POINT('',(19.39,-7.8,-52.11));
#21742=CARTESIAN_POINT('',(19.,-7.41,-52.11));
#21743=CARTESIAN_POINT('Origin',(26.5,-7.605,-52.305));
#21744=CARTESIAN_POINT('',(26.5,-7.8,-52.11));
#21745=CARTESIAN_POINT('',(26.5,-7.41,-52.5));
#21746=CARTESIAN_POINT('Origin',(19.39,-7.41,-42.5));
#21747=CARTESIAN_POINT('',(19.39,-7.8,-42.89));
#21748=CARTESIAN_POINT('',(19.,-7.41,-42.89));
#21749=CARTESIAN_POINT('',(19.39,-7.8,-42.89));
#21750=CARTESIAN_POINT('',(19.39,-7.41,-42.5));
#21751=CARTESIAN_POINT('',(19.39,-7.41,-42.5));
#21752=CARTESIAN_POINT('',(19.,-7.41,-42.89));
#21753=CARTESIAN_POINT('Origin',(21.5,-7.605,-42.695));
#21754=CARTESIAN_POINT('',(21.5,-7.8,-42.89));
#21755=CARTESIAN_POINT('',(21.5,-7.41,-42.5));
#21756=CARTESIAN_POINT('Origin',(19.195,-7.8,-42.695));
#21757=CARTESIAN_POINT('',(19.,-7.8,-42.89));
#21758=CARTESIAN_POINT('',(19.39,-7.8,-42.5));
#21759=CARTESIAN_POINT('Origin',(19.195,-7.605,-50.));
#21760=CARTESIAN_POINT('',(19.39,-7.8,-50.));
#21761=CARTESIAN_POINT('',(19.,-7.41,-50.));
#21762=CARTESIAN_POINT('Origin',(19.195,-7.8,-52.305));
#21763=CARTESIAN_POINT('',(19.39,-7.8,-52.5));
#21764=CARTESIAN_POINT('',(19.,-7.8,-52.11));
#21765=CARTESIAN_POINT('Origin',(21.5,1.805,-42.695));
#21766=CARTESIAN_POINT('',(21.5,2.,-42.89));
#21767=CARTESIAN_POINT('',(21.5,1.61,-42.5));
#21768=CARTESIAN_POINT('Origin',(19.195,1.805,-50.));
#21769=CARTESIAN_POINT('',(19.39,2.,-50.));
#21770=CARTESIAN_POINT('',(19.,1.61,-50.));
#21771=CARTESIAN_POINT('Origin',(28.805,-7.605,-45.));
#21772=CARTESIAN_POINT('',(28.61,-7.8,-45.));
#21773=CARTESIAN_POINT('',(29.,-7.41,-45.));
#21774=CARTESIAN_POINT('Origin',(28.805,-7.8,-42.695));
#21775=CARTESIAN_POINT('',(28.61,-7.8,-42.5));
#21776=CARTESIAN_POINT('',(29.,-7.8,-42.89));
#21777=CARTESIAN_POINT('Origin',(26.5,1.805,-52.305));
#21778=CARTESIAN_POINT('',(26.5,2.,-52.11));
#21779=CARTESIAN_POINT('',(26.5,1.61,-52.5));
#21780=CARTESIAN_POINT('Origin',(28.805,-7.8,-52.305));
#21781=CARTESIAN_POINT('',(29.,-7.8,-52.11));
#21782=CARTESIAN_POINT('',(28.61,-7.8,-52.5));
#21783=CARTESIAN_POINT('Origin',(28.805,1.805,-45.));
#21784=CARTESIAN_POINT('',(28.61,2.,-45.));
#21785=CARTESIAN_POINT('',(29.,1.61,-45.));
#21786=CARTESIAN_POINT('Origin',(29.,-7.8,-52.5));
#21787=CARTESIAN_POINT('Origin',(19.,-7.8,-42.5));
#21788=CARTESIAN_POINT('Origin',(24.,-7.8,-47.5));
#21789=CARTESIAN_POINT('',(19.95,-7.8,-47.5));
#21790=CARTESIAN_POINT('Origin',(24.,-7.8,-47.5));
#21791=CARTESIAN_POINT('Origin',(19.,-7.8,-52.5));
#21792=CARTESIAN_POINT('Origin',(24.,2.,-47.5));
#21793=CARTESIAN_POINT('',(19.95,2.,-47.5));
#21794=CARTESIAN_POINT('Origin',(24.,2.,-47.5));
#21795=CARTESIAN_POINT('Origin',(29.,-7.8,-42.5));
#21796=CARTESIAN_POINT('Origin',(24.,2.,-47.5));
#21797=CARTESIAN_POINT('',(19.95,2.,-47.5));
#37158=UNCERTAINTY_MEASURE_WITH_UNIT(LENGTH_MEASURE(0.01),#37182,
'DISTANCE_ACCURACY_VALUE',
'Maximum model space distance between geometric entities at asserted c
onnectivities');
#37166=UNCERTAINTY_MEASURE_WITH_UNIT(LENGTH_MEASURE(0.01),#37182,
'DISTANCE_ACCURACY_VALUE',
'Maximum model space distance between geometric entities at asserted c
onnectivities');
#37173=(
GEOMETRIC_REPRESENTATION_CONTEXT(3)
GLOBAL_UNCERTAINTY_ASSIGNED_CONTEXT((#37158))
GLOBAL_UNIT_ASSIGNED_CONTEXT((#37182,#37184,#37185))
REPRESENTATION_CONTEXT('','3D')
);
#37181=(
GEOMETRIC_REPRESENTATION_CONTEXT(3)
GLOBAL_UNCERTAINTY_ASSIGNED_CONTEXT((#37166))
GLOBAL_UNIT_ASSIGNED_CONTEXT((#37182,#37184,#37185))
REPRESENTATION_CONTEXT('','3D')
);
#37182=(
LENGTH_UNIT()
NAMED_UNIT(*)
SI_UNIT(.MILLI.,.METRE.)
);
#37184=(
NAMED_UNIT(*)
PLANE_ANGLE_UNIT()
SI_UNIT($,.RADIAN.)
);
#37185=(
NAMED_UNIT(*)
SI_UNIT($,.STERADIAN.)
SOLID_ANGLE_UNIT()
);
#37192=SHAPE_DEFINITION_REPRESENTATION(#37206,#37243);
#37206=PRODUCT_DEFINITION_SHAPE('',$,#37258);
#37243=SHAPE_REPRESENTATION('',(#15425),#37173);
#37251=PRODUCT_DEFINITION_CONTEXT('part definition',#37295,'design');
#37258=PRODUCT_DEFINITION('2026-10-20-13-23-55-996','06_M8_Lens_Holder',
#37272,#37251);
#37272=PRODUCT_DEFINITION_FORMATION('',$,#37303);
#37295=APPLICATION_CONTEXT(
'Core Data for Automotive Mechanical Design Process');
#37296=PRODUCT_CONTEXT('part definition',#37295,'mechanical');
#37303=PRODUCT('2026-10-20-13-23-55-996','06_M8_Lens_Holder',$,(#37296));
#37360=COLOUR_RGB('Sky Blue',0.24,0.69,0.87);
#37361=FILL_AREA_STYLE_COLOUR('',#37360);
#37362=FILL_AREA_STYLE('',(#37361));
#37363=SURFACE_STYLE_FILL_AREA(#37362);
#37364=SURFACE_SIDE_STYLE('',(#37363));
#37365=SURFACE_STYLE_USAGE(.BOTH.,#37364);
#37366=PRESENTATION_STYLE_ASSIGNMENT((#37365));
ENDSEC;
END-ISO-10303-21;
